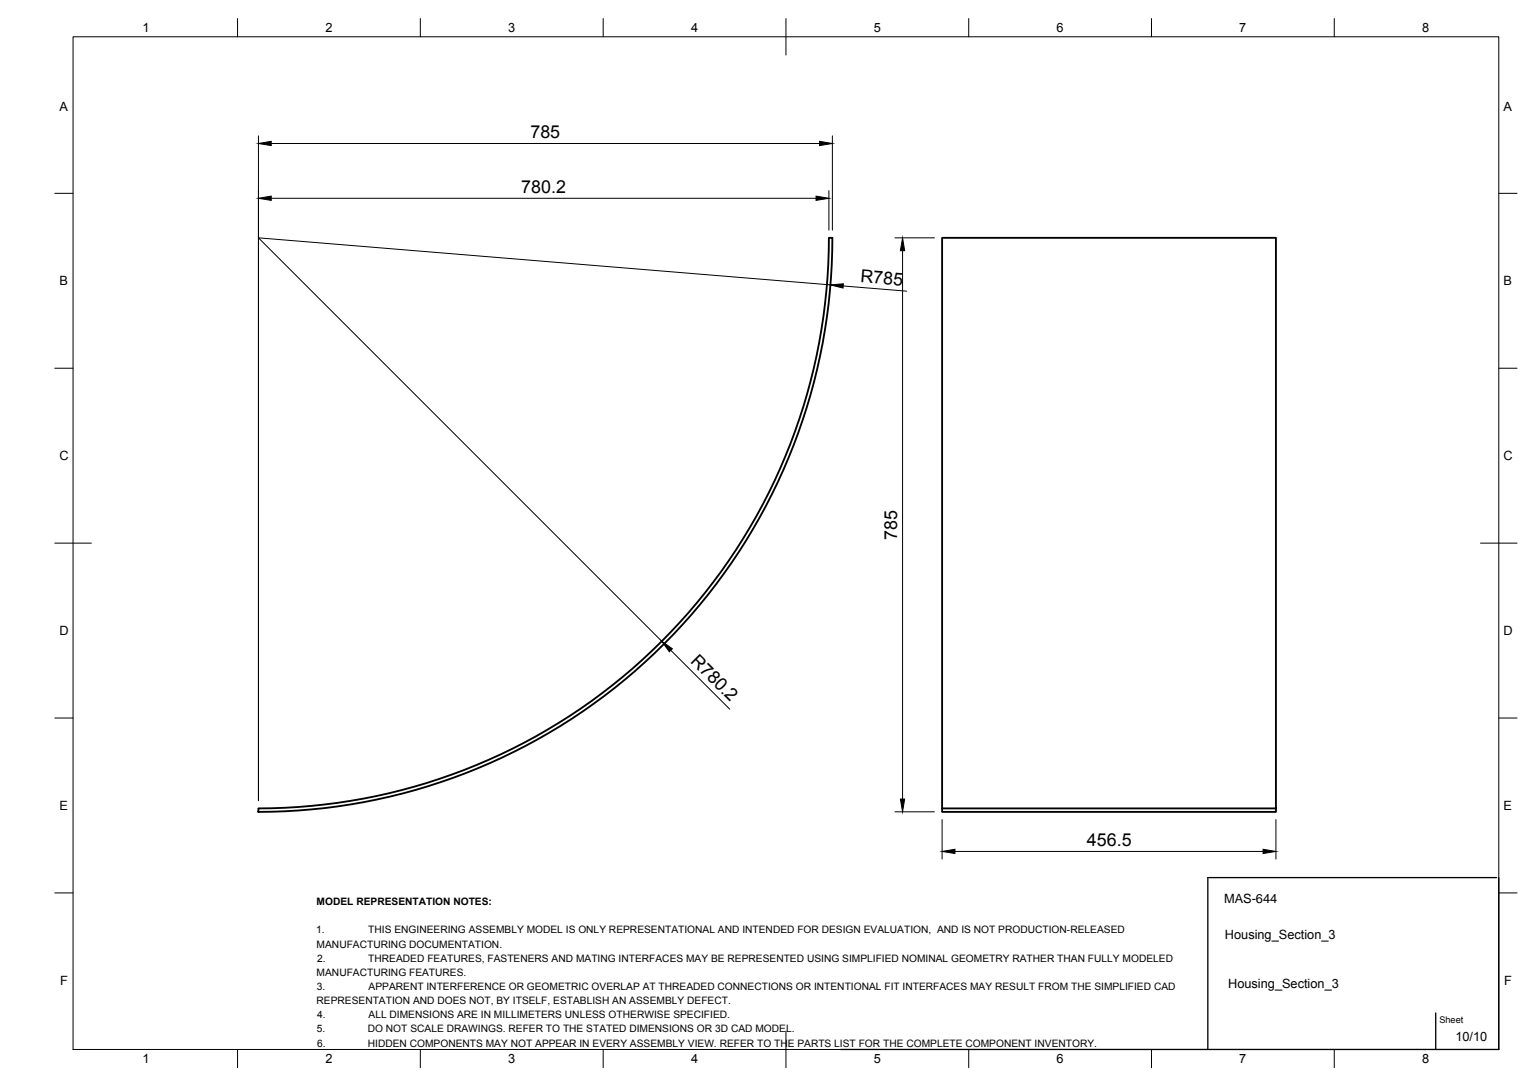
ISO-10303-21;
HEADER;
FILE_DESCRIPTION((''),'2;1');
FILE_NAME('Housing_Section_3.step','2026-10-09T11:38:21-07:00',(''),(''),'','','');
FILE_SCHEMA (('AUTOMOTIVE_DESIGN { 1 0 10303 214 3 1 1 }'));
ENDSEC;
DATA;
#10=MECHANICAL_DESIGN_GEOMETRIC_PRESENTATION_REPRESENTATION('',(#66),#3619);
#50=SHAPE_REPRESENTATION_RELATIONSHIP('SRR','None',#3658,#58) ;
#58=ADVANCED_BREP_SHAPE_REPRESENTATION('',(#74),#3618) ;
#66=STYLED_ITEM('',(#3700),#74) ;
#74=MANIFOLD_SOLID_BREP('Body1',#2090) ;
#209=PLANE('',#2394) ;
#210=PLANE('',#2398) ;
#211=PLANE('',#2399) ;
#212=PLANE('',#2400) ;
#315=FACE_OUTER_BOUND('',#505,.T.) ;
#316=FACE_OUTER_BOUND('',#506,.T.) ;
#317=FACE_OUTER_BOUND('',#507,.T.) ;
#318=FACE_OUTER_BOUND('',#508,.T.) ;
#319=FACE_OUTER_BOUND('',#509,.T.) ;
#320=FACE_OUTER_BOUND('',#510,.T.) ;
#505=EDGE_LOOP('',(#1899,#1900,#1901,#1902)) ;
#506=EDGE_LOOP('',(#1903,#1904,#1905,#1906)) ;
#507=EDGE_LOOP('',(#1907,#1908,#1909,#1910)) ;
#508=EDGE_LOOP('',(#1911,#1912,#1913,#1914)) ;
#509=EDGE_LOOP('',(#1915,#1916,#1917,#1918)) ;
#510=EDGE_LOOP('',(#1919,#1920,#1921,#1922)) ;
#667=LINE('',#3571,#831) ;
#668=LINE('',#3574,#832) ;
#669=LINE('',#3577,#833) ;
#670=LINE('',#3579,#834) ;
#671=LINE('',#3580,#835) ;
#672=LINE('',#3585,#836) ;
#673=LINE('',#3588,#837) ;
#674=LINE('',#3589,#838) ;
#831=VECTOR('',#2991,1000.) ;
#832=VECTOR('',#2994,1000.) ;
#833=VECTOR('',#2997,1000.) ;
#834=VECTOR('',#2998,1000.) ;
#835=VECTOR('',#2999,1000.) ;
#836=VECTOR('',#3004,1000.) ;
#837=VECTOR('',#3009,1000.) ;
#838=VECTOR('',#3010,1000.) ;
#939=CIRCLE('',#2392,780.2) ;
#940=CIRCLE('',#2393,780.2) ;
#941=CIRCLE('',#2396,785.) ;
#942=CIRCLE('',#2397,785.) ;
#1111=VERTEX_POINT('',#3567) ;
#1112=VERTEX_POINT('',#3568) ;
#1113=VERTEX_POINT('',#3570) ;
#1114=VERTEX_POINT('',#3572) ;
#1115=VERTEX_POINT('',#3576) ;
#1116=VERTEX_POINT('',#3578) ;
#1117=VERTEX_POINT('',#3582) ;
#1118=VERTEX_POINT('',#3584) ;
#1375=EDGE_CURVE('',#1111,#1112,#939,.T.) ;
#1376=EDGE_CURVE('',#1113,#1112,#667,.T.) ;
#1377=EDGE_CURVE('',#1114,#1113,#940,.T.) ;
#1378=EDGE_CURVE('',#1114,#1111,#668,.T.) ;
#1379=EDGE_CURVE('',#1115,#1112,#669,.T.) ;
#1380=EDGE_CURVE('',#1116,#1115,#670,.T.) ;
#1381=EDGE_CURVE('',#1116,#1113,#671,.T.) ;
#1382=EDGE_CURVE('',#1117,#1115,#941,.T.) ;
#1383=EDGE_CURVE('',#1118,#1117,#672,.T.) ;
#1384=EDGE_CURVE('',#1118,#1116,#942,.T.) ;
#1385=EDGE_CURVE('',#1111,#1117,#673,.T.) ;
#1386=EDGE_CURVE('',#1114,#1118,#674,.T.) ;
#1899=ORIENTED_EDGE('',*,*,#1375,.T.) ;
#1900=ORIENTED_EDGE('',*,*,#1376,.F.) ;
#1901=ORIENTED_EDGE('',*,*,#1377,.F.) ;
#1902=ORIENTED_EDGE('',*,*,#1378,.T.) ;
#1903=ORIENTED_EDGE('',*,*,#1379,.F.) ;
#1904=ORIENTED_EDGE('',*,*,#1380,.F.) ;
#1905=ORIENTED_EDGE('',*,*,#1381,.T.) ;
#1906=ORIENTED_EDGE('',*,*,#1376,.T.) ;
#1907=ORIENTED_EDGE('',*,*,#1382,.F.) ;
#1908=ORIENTED_EDGE('',*,*,#1383,.F.) ;
#1909=ORIENTED_EDGE('',*,*,#1384,.T.) ;
#1910=ORIENTED_EDGE('',*,*,#1380,.T.) ;
#1911=ORIENTED_EDGE('',*,*,#1385,.F.) ;
#1912=ORIENTED_EDGE('',*,*,#1378,.F.) ;
#1913=ORIENTED_EDGE('',*,*,#1386,.T.) ;
#1914=ORIENTED_EDGE('',*,*,#1383,.T.) ;
#1915=ORIENTED_EDGE('',*,*,#1377,.T.) ;
#1916=ORIENTED_EDGE('',*,*,#1381,.F.) ;
#1917=ORIENTED_EDGE('',*,*,#1384,.F.) ;
#1918=ORIENTED_EDGE('',*,*,#1386,.F.) ;
#1919=ORIENTED_EDGE('',*,*,#1375,.F.) ;
#1920=ORIENTED_EDGE('',*,*,#1385,.T.) ;
#1921=ORIENTED_EDGE('',*,*,#1382,.T.) ;
#1922=ORIENTED_EDGE('',*,*,#1379,.T.) ;
#1973=CYLINDRICAL_SURFACE('',#2391,780.2) ;
#1974=CYLINDRICAL_SURFACE('',#2395,785.) ;
#2077=ADVANCED_FACE('',(#315),#1973,.F.) ;
#2078=ADVANCED_FACE('',(#316),#209,.T.) ;
#2079=ADVANCED_FACE('',(#317),#1974,.T.) ;
#2080=ADVANCED_FACE('',(#318),#210,.T.) ;
#2081=ADVANCED_FACE('',(#319),#211,.T.) ;
#2082=ADVANCED_FACE('',(#320),#212,.F.) ;
#2090=CLOSED_SHELL('',(#2077,#2078,#2079,#2080,#2081,#2082)) ;
#2390=AXIS2_PLACEMENT_3D('',#3565,#2985,#2986) ;
#2391=AXIS2_PLACEMENT_3D('',#3566,#2987,#2988) ;
#2392=AXIS2_PLACEMENT_3D('',#3569,#2989,#2990) ;
#2393=AXIS2_PLACEMENT_3D('',#3573,#2992,#2993) ;
#2394=AXIS2_PLACEMENT_3D('',#3575,#2995,#2996) ;
#2395=AXIS2_PLACEMENT_3D('',#3581,#3000,#3001) ;
#2396=AXIS2_PLACEMENT_3D('',#3583,#3002,#3003) ;
#2397=AXIS2_PLACEMENT_3D('',#3586,#3005,#3006) ;
#2398=AXIS2_PLACEMENT_3D('',#3587,#3007,#3008) ;
#2399=AXIS2_PLACEMENT_3D('',#3590,#3011,#3012) ;
#2400=AXIS2_PLACEMENT_3D('',#3591,#3013,#3014) ;
#2985=DIRECTION('axis',(0.,0.,1.)) ;
#2986=DIRECTION('refdir',(1.,0.,0.)) ;
#2987=DIRECTION('center_axis',(2.50028956146539E-17,2.89689231211468E-18,
1.)) ;
#2988=DIRECTION('ref_axis',(1.,-8.74300631892311E-16,-2.50028956146539E-17)) ;
#2989=DIRECTION('center_axis',(2.50028956146539E-17,2.89689231211468E-18,
1.)) ;
#2990=DIRECTION('ref_axis',(-1.,8.74300631892311E-16,2.50028956146539E-17)) ;
#2991=DIRECTION('',(2.50028956146539E-17,2.89689231211468E-18,1.)) ;
#2992=DIRECTION('center_axis',(2.50028956146539E-17,2.89689231211468E-18,
1.)) ;
#2993=DIRECTION('ref_axis',(-1.,8.74300631892311E-16,2.50028956146539E-17)) ;
#2994=DIRECTION('',(2.50028956146539E-17,2.89689231211468E-18,1.)) ;
#2995=DIRECTION('center_axis',(1.,-6.07748371951869E-14,-2.50028956146538E-17)) ;
#2996=DIRECTION('ref_axis',(-6.07748371951869E-14,-1.,2.8968923121162E-18)) ;
#2997=DIRECTION('',(6.07748371951869E-14,1.,-2.8968923121162E-18)) ;
#2998=DIRECTION('',(2.50028956146539E-17,2.89689231211468E-18,1.)) ;
#2999=DIRECTION('',(6.07748371951869E-14,1.,-2.8968923121162E-18)) ;
#3000=DIRECTION('center_axis',(2.50028956146539E-17,2.89689231211468E-18,
1.)) ;
#3001=DIRECTION('ref_axis',(1.,-8.74300631892311E-16,-2.50028956146539E-17)) ;
#3002=DIRECTION('center_axis',(2.50028956146539E-17,2.89689231211468E-18,
1.)) ;
#3003=DIRECTION('ref_axis',(1.,-8.74300631892311E-16,-2.50028956146539E-17)) ;
#3004=DIRECTION('',(2.50028956146539E-17,2.89689231211468E-18,1.)) ;
#3005=DIRECTION('center_axis',(2.50028956146539E-17,2.89689231211468E-18,
1.)) ;
#3006=DIRECTION('ref_axis',(1.,-8.74300631892311E-16,-2.50028956146539E-17)) ;
#3007=DIRECTION('center_axis',(9.96765311807047E-16,1.,-2.8968923121147E-18)) ;
#3008=DIRECTION('ref_axis',(1.,-9.96765311807047E-16,-2.50028956146539E-17)) ;
#3009=DIRECTION('',(-1.,9.96765311807047E-16,2.50028956146539E-17)) ;
#3010=DIRECTION('',(-1.,9.96765311807047E-16,2.50028956146539E-17)) ;
#3011=DIRECTION('center_axis',(-2.50028956146539E-17,-2.89689231211468E-18,
-1.)) ;
#3012=DIRECTION('ref_axis',(-1.,8.74300631892311E-16,2.50028956146539E-17)) ;
#3013=DIRECTION('center_axis',(-2.50028956146539E-17,-2.89689231211468E-18,
-1.)) ;
#3014=DIRECTION('ref_axis',(-1.,8.74300631892311E-16,2.50028956146539E-17)) ;
#3565=CARTESIAN_POINT('',(0.,0.,0.)) ;
#3566=CARTESIAN_POINT('Origin',(99.9999999999999,1.35042597812193E-13,4.44089209850063E-13)) ;
#3567=CARTESIAN_POINT('',(-680.2,9.14041325424531E-13,456.5)) ;
#3568=CARTESIAN_POINT('',(99.9999999999994,-780.2,456.5)) ;
#3569=CARTESIAN_POINT('Origin',(99.9999999999999,1.36365029152673E-13,456.5)) ;
#3570=CARTESIAN_POINT('',(99.9999999999993,-780.2,4.44089209850063E-13)) ;
#3571=CARTESIAN_POINT('',(99.9999999999993,-780.2,4.44089209850063E-13)) ;
#3572=CARTESIAN_POINT('',(-680.2,9.1271889408405E-13,4.71844785465692E-13)) ;
#3573=CARTESIAN_POINT('Origin',(99.9999999999999,1.35042597812193E-13,4.44089209850063E-13)) ;
#3574=CARTESIAN_POINT('',(-680.2,9.1271889408405E-13,4.71844785465692E-13)) ;
#3575=CARTESIAN_POINT('Origin',(99.999999999999,-785.,4.44089209850063E-13)) ;
#3576=CARTESIAN_POINT('',(99.9999999999991,-785.,456.5)) ;
#3577=CARTESIAN_POINT('',(99.9999999999991,-785.,456.5)) ;
#3578=CARTESIAN_POINT('',(99.999999999999,-785.,4.44089209850063E-13)) ;
#3579=CARTESIAN_POINT('',(99.999999999999,-785.,4.44089209850063E-13)) ;
#3580=CARTESIAN_POINT('',(99.999999999999,-785.,4.44089209850063E-13)) ;
#3581=CARTESIAN_POINT('Origin',(99.9999999999999,1.35042597812193E-13,4.44089209850063E-13)) ;
#3582=CARTESIAN_POINT('',(-685.,9.18825798921204E-13,456.5)) ;
#3583=CARTESIAN_POINT('Origin',(99.9999999999999,1.36365029152673E-13,456.5)) ;
#3584=CARTESIAN_POINT('',(-685.,9.17503367580724E-13,4.71844785465692E-13)) ;
#3585=CARTESIAN_POINT('',(-685.,9.17503367580724E-13,4.71844785465692E-13)) ;
#3586=CARTESIAN_POINT('Origin',(99.9999999999999,1.35042597812193E-13,4.44089209850063E-13)) ;
#3587=CARTESIAN_POINT('Origin',(-680.2,9.1271889408405E-13,4.71844785465692E-13)) ;
#3588=CARTESIAN_POINT('',(-680.2,9.14041325424531E-13,456.5)) ;
#3589=CARTESIAN_POINT('',(-680.2,9.1271889408405E-13,4.71844785465692E-13)) ;
#3590=CARTESIAN_POINT('Origin',(99.9999999999999,1.35042597812193E-13,4.44089209850063E-13)) ;
#3591=CARTESIAN_POINT('Origin',(99.9999999999999,1.36365029152673E-13,456.5)) ;
#3608=UNCERTAINTY_MEASURE_WITH_UNIT(LENGTH_MEASURE(0.01),#3620,
'DISTANCE_ACCURACY_VALUE',
'Maximum model space distance between geometric entities at asserted c
onnectivities') ;
#3609=UNCERTAINTY_MEASURE_WITH_UNIT(LENGTH_MEASURE(0.01),#3620,
'DISTANCE_ACCURACY_VALUE',
'Maximum model space distance between geometric entities at asserted c
onnectivities') ;
#3618=(
GEOMETRIC_REPRESENTATION_CONTEXT(3)
GLOBAL_UNCERTAINTY_ASSIGNED_CONTEXT((#3608))
GLOBAL_UNIT_ASSIGNED_CONTEXT((#3620,#3622,#3623))
REPRESENTATION_CONTEXT('','3D')
) ;
#3619=(
GEOMETRIC_REPRESENTATION_CONTEXT(3)
GLOBAL_UNCERTAINTY_ASSIGNED_CONTEXT((#3609))
GLOBAL_UNIT_ASSIGNED_CONTEXT((#3620,#3622,#3623))
REPRESENTATION_CONTEXT('','3D')
) ;
#3620=(
LENGTH_UNIT()
NAMED_UNIT(*)
SI_UNIT(.MILLI.,.METRE.)
) ;
#3622=(
NAMED_UNIT(*)
PLANE_ANGLE_UNIT()
SI_UNIT($,.RADIAN.)
) ;
#3623=(
NAMED_UNIT(*)
SI_UNIT($,.STERADIAN.)
SOLID_ANGLE_UNIT()
) ;
#3632=SHAPE_DEFINITION_REPRESENTATION(#3641,#3658) ;
#3641=PRODUCT_DEFINITION_SHAPE('',$,#3668) ;
#3658=SHAPE_REPRESENTATION('',(#2390),#3618) ;
#3659=PRODUCT_DEFINITION_CONTEXT('part definition',#3688,'design') ;
#3668=PRODUCT_DEFINITION('Housing_Section_3','Housing_Section_3',#3677,
#3659) ;
#3677=PRODUCT_DEFINITION_FORMATION('',$,#3698) ;
#3688=APPLICATION_CONTEXT(
'Core Data for Automotive Mechanical Design Process') ;
#3689=PRODUCT_CONTEXT('part definition',#3688,'mechanical') ;
#3698=PRODUCT('Housing_Section_3','Housing_Section_3',$,(#3689)) ;
#3700=PRESENTATION_STYLE_ASSIGNMENT((#3702)) ;
#3702=SURFACE_STYLE_USAGE(.BOTH.,#3704) ;
#3704=SURFACE_SIDE_STYLE('',(#3706)) ;
#3706=SURFACE_STYLE_FILL_AREA(#3708) ;
#3708=FILL_AREA_STYLE('Opaque(202,209,238)',(#3710)) ;
#3710=FILL_AREA_STYLE_COLOUR('Opaque(202,209,238)',#3712) ;
#3712=COLOUR_RGB('Opaque(202,209,238)', 0.09019608, 0.27058824, 0.51372549) ;
ENDSEC;
END-ISO-10303-21;
